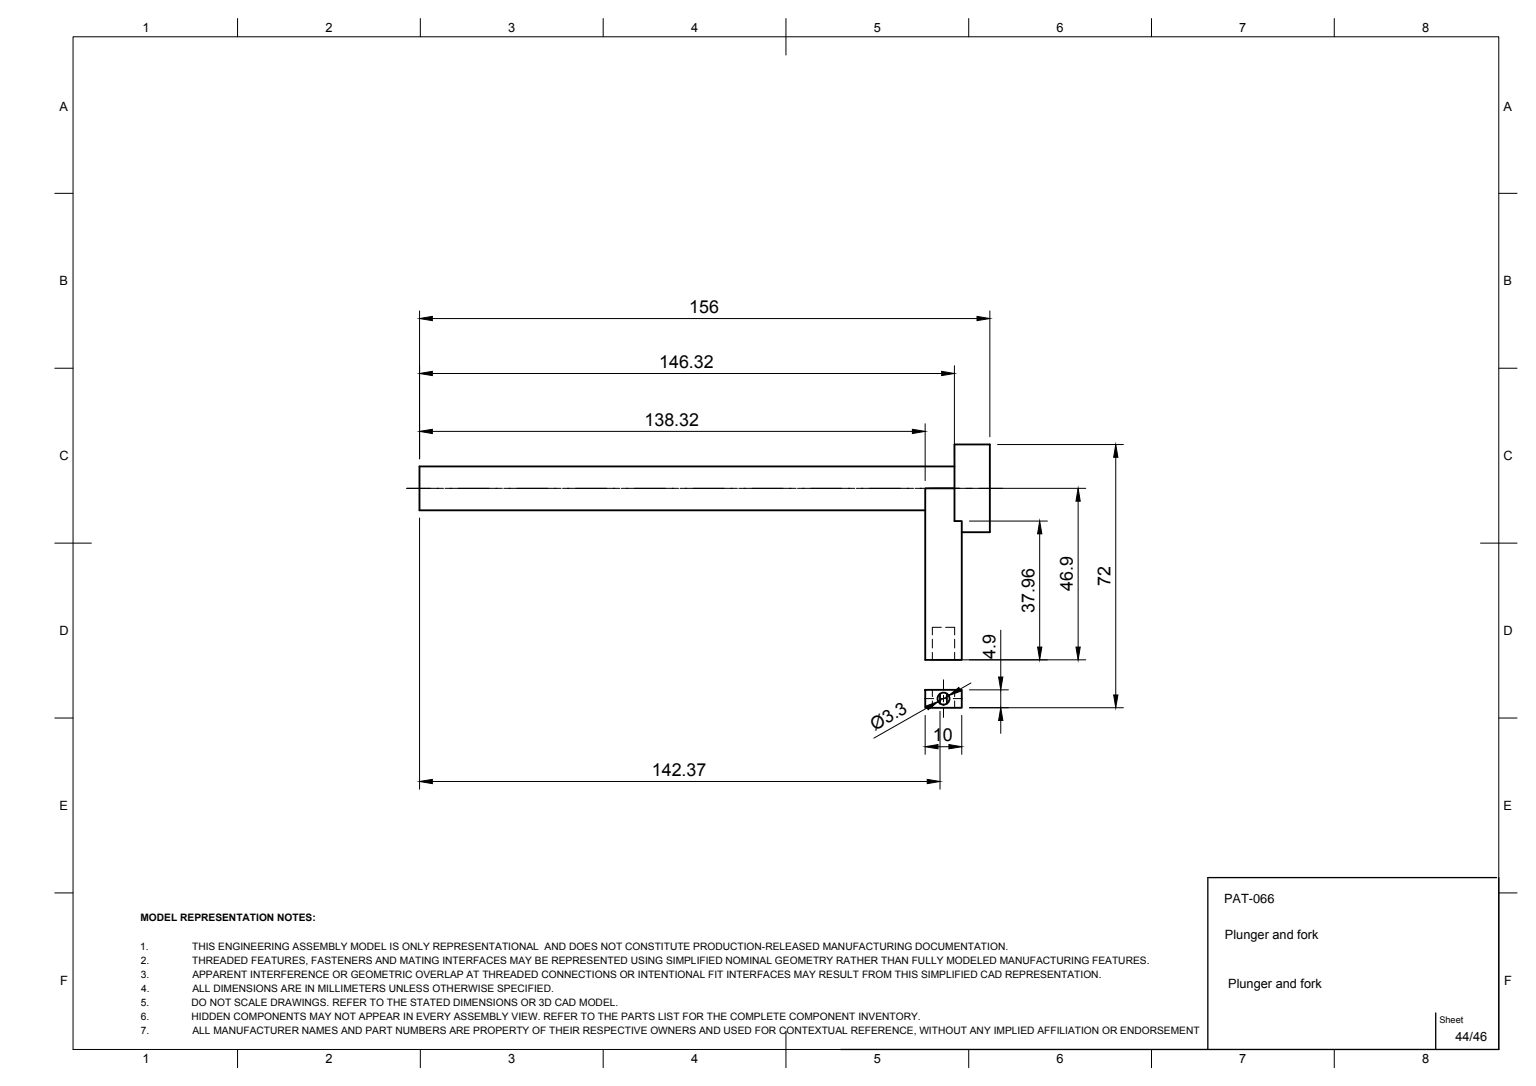
ISO-10303-21;
HEADER;
/* Generated by software containing ST-Developer
 * from STEP Tools, Inc. (www.steptools.com) 
 */

FILE_DESCRIPTION(
/* description */ ('Lever-operated bar clamp (toggle)'),
/* implementation_level */ '2;1');

FILE_NAME(
/* name */ 'Plunger and fork.step',
/* time_stamp */ '2026-10-28T03:25:02-07:00',
/* author */ (''),
/* organization */ (''),
/* preprocessor_version */ 'ST-DEVELOPER v20.2',
/* originating_system */ 'Autodesk Translation Framework v15.17.0.0',
/* authorisation */ '');

FILE_SCHEMA (('AUTOMOTIVE_DESIGN { 1 0 10303 214 3 1 1 }'));
ENDSEC;

DATA;
#10=MECHANICAL_DESIGN_GEOMETRIC_PRESENTATION_REPRESENTATION('',(#452,#453),#12413);
#285=B_SPLINE_CURVE_WITH_KNOTS('',3,(#12174,#12175,#12176,#12177,#12178,
#12179,#12180,#12181,#12182,#12183),.UNSPECIFIED.,.F.,.F.,(4,2,2,2,4),(0.66642709076087,
0.700624974512804,0.764181514210609,0.827738053908413,0.861935937660348),
 .UNSPECIFIED.);
#286=B_SPLINE_CURVE_WITH_KNOTS('',3,(#12191,#12192,#12193,#12194,#12195,
#12196,#12197,#12198,#12199,#12200),.UNSPECIFIED.,.F.,.F.,(4,2,2,2,4),(0.156972747953797,
0.191170631705732,0.254727171403536,0.318283711101341,0.352481594853276),
 .UNSPECIFIED.);
#368=SHAPE_REPRESENTATION_RELATIONSHIP('SRR','None',#12612,#406);
#406=ADVANCED_BREP_SHAPE_REPRESENTATION('',(#495,#496),#12409);
#452=STYLED_ITEM('',(#12883),#495);
#453=STYLED_ITEM('',(#12883),#496);
#495=MANIFOLD_SOLID_BREP('Body1',#6615);
#496=MANIFOLD_SOLID_BREP('Body2',#6616);
#644=FACE_BOUND('',#1803,.T.);
#645=FACE_BOUND('',#1819,.T.);
#646=FACE_BOUND('',#1821,.T.);
#647=FACE_BOUND('',#1826,.T.);
#648=FACE_BOUND('',#1828,.T.);
#855=PLANE('',#7817);
#856=PLANE('',#7818);
#857=PLANE('',#7819);
#858=PLANE('',#7820);
#859=PLANE('',#7822);
#860=PLANE('',#7823);
#861=PLANE('',#7824);
#862=PLANE('',#7825);
#863=PLANE('',#7830);
#864=PLANE('',#7835);
#865=PLANE('',#7836);
#866=PLANE('',#7837);
#867=PLANE('',#7843);
#868=PLANE('',#7847);
#869=PLANE('',#7848);
#870=PLANE('',#7849);
#871=PLANE('',#7850);
#872=PLANE('',#7851);
#873=PLANE('',#7852);
#1250=FACE_OUTER_BOUND('',#1800,.T.);
#1251=FACE_OUTER_BOUND('',#1801,.T.);
#1252=FACE_OUTER_BOUND('',#1802,.T.);
#1253=FACE_OUTER_BOUND('',#1804,.T.);
#1254=FACE_OUTER_BOUND('',#1805,.T.);
#1255=FACE_OUTER_BOUND('',#1806,.T.);
#1256=FACE_OUTER_BOUND('',#1807,.T.);
#1257=FACE_OUTER_BOUND('',#1808,.T.);
#1258=FACE_OUTER_BOUND('',#1809,.T.);
#1259=FACE_OUTER_BOUND('',#1810,.T.);
#1260=FACE_OUTER_BOUND('',#1811,.T.);
#1261=FACE_OUTER_BOUND('',#1812,.T.);
#1262=FACE_OUTER_BOUND('',#1813,.T.);
#1263=FACE_OUTER_BOUND('',#1814,.T.);
#1264=FACE_OUTER_BOUND('',#1815,.T.);
#1265=FACE_OUTER_BOUND('',#1816,.T.);
#1266=FACE_OUTER_BOUND('',#1817,.T.);
#1267=FACE_OUTER_BOUND('',#1818,.T.);
#1268=FACE_OUTER_BOUND('',#1820,.T.);
#1269=FACE_OUTER_BOUND('',#1822,.T.);
#1270=FACE_OUTER_BOUND('',#1823,.T.);
#1271=FACE_OUTER_BOUND('',#1824,.T.);
#1272=FACE_OUTER_BOUND('',#1825,.T.);
#1273=FACE_OUTER_BOUND('',#1827,.T.);
#1800=EDGE_LOOP('',(#5853,#5854,#5855,#5856));
#1801=EDGE_LOOP('',(#5857));
#1802=EDGE_LOOP('',(#5858,#5859,#5860,#5861));
#1803=EDGE_LOOP('',(#5862));
#1804=EDGE_LOOP('',(#5863,#5864,#5865,#5866,#5867,#5868));
#1805=EDGE_LOOP('',(#5869,#5870,#5871,#5872));
#1806=EDGE_LOOP('',(#5873,#5874,#5875,#5876,#5877,#5878));
#1807=EDGE_LOOP('',(#5879,#5880,#5881,#5882));
#1808=EDGE_LOOP('',(#5883,#5884,#5885,#5886));
#1809=EDGE_LOOP('',(#5887,#5888,#5889,#5890,#5891,#5892));
#1810=EDGE_LOOP('',(#5893,#5894,#5895,#5896,#5897,#5898,#5899));
#1811=EDGE_LOOP('',(#5900,#5901,#5902,#5903,#5904,#5905,#5906));
#1812=EDGE_LOOP('',(#5907,#5908,#5909,#5910,#5911,#5912,#5913,#5914));
#1813=EDGE_LOOP('',(#5915));
#1814=EDGE_LOOP('',(#5916));
#1815=EDGE_LOOP('',(#5917,#5918));
#1816=EDGE_LOOP('',(#5919,#5920,#5921,#5922,#5923,#5924,#5925,#5926));
#1817=EDGE_LOOP('',(#5927,#5928,#5929));
#1818=EDGE_LOOP('',(#5930,#5931,#5932,#5933));
#1819=EDGE_LOOP('',(#5934,#5935,#5936,#5937));
#1820=EDGE_LOOP('',(#5938,#5939,#5940,#5941));
#1821=EDGE_LOOP('',(#5942));
#1822=EDGE_LOOP('',(#5943,#5944,#5945,#5946));
#1823=EDGE_LOOP('',(#5947,#5948,#5949,#5950));
#1824=EDGE_LOOP('',(#5951,#5952,#5953,#5954));
#1825=EDGE_LOOP('',(#5955,#5956,#5957,#5958));
#1826=EDGE_LOOP('',(#5959));
#1827=EDGE_LOOP('',(#5960,#5961,#5962,#5963));
#1828=EDGE_LOOP('',(#5964));
#2229=LINE('',#12104,#2670);
#2230=LINE('',#12110,#2671);
#2231=LINE('',#12112,#2672);
#2232=LINE('',#12114,#2673);
#2233=LINE('',#12115,#2674);
#2234=LINE('',#12118,#2675);
#2235=LINE('',#12120,#2676);
#2236=LINE('',#12122,#2677);
#2237=LINE('',#12124,#2678);
#2238=LINE('',#12125,#2679);
#2239=LINE('',#12128,#2680);
#2240=LINE('',#12132,#2681);
#2241=LINE('',#12134,#2682);
#2242=LINE('',#12136,#2683);
#2243=LINE('',#12137,#2684);
#2244=LINE('',#12141,#2685);
#2245=LINE('',#12142,#2686);
#2246=LINE('',#12143,#2687);
#2247=LINE('',#12146,#2688);
#2248=LINE('',#12148,#2689);
#2249=LINE('',#12149,#2690);
#2250=LINE('',#12155,#2691);
#2251=LINE('',#12163,#2692);
#2252=LINE('',#12170,#2693);
#2253=LINE('',#12187,#2694);
#2254=LINE('',#12202,#2695);
#2255=LINE('',#12207,#2696);
#2256=LINE('',#12212,#2697);
#2257=LINE('',#12214,#2698);
#2258=LINE('',#12216,#2699);
#2259=LINE('',#12217,#2700);
#2260=LINE('',#12221,#2701);
#2261=LINE('',#12222,#2702);
#2262=LINE('',#12223,#2703);
#2263=LINE('',#12226,#2704);
#2264=LINE('',#12227,#2705);
#2265=LINE('',#12230,#2706);
#2266=LINE('',#12231,#2707);
#2267=LINE('',#12233,#2708);
#2670=VECTOR('',#9826,0.305);
#2671=VECTOR('',#9833,1.);
#2672=VECTOR('',#9834,1.);
#2673=VECTOR('',#9835,1.);
#2674=VECTOR('',#9836,1.);
#2675=VECTOR('',#9839,1.);
#2676=VECTOR('',#9840,1.);
#2677=VECTOR('',#9841,1.);
#2678=VECTOR('',#9842,1.);
#2679=VECTOR('',#9843,1.);
#2680=VECTOR('',#9846,1.);
#2681=VECTOR('',#9851,1.);
#2682=VECTOR('',#9852,1.);
#2683=VECTOR('',#9853,1.);
#2684=VECTOR('',#9854,1.);
#2685=VECTOR('',#9857,1.);
#2686=VECTOR('',#9858,1.);
#2687=VECTOR('',#9859,1.);
#2688=VECTOR('',#9862,1.);
#2689=VECTOR('',#9863,1.);
#2690=VECTOR('',#9864,1.);
#2691=VECTOR('',#9873,0.6);
#2692=VECTOR('',#9884,1.2);
#2693=VECTOR('',#9893,1.);
#2694=VECTOR('',#9900,0.165);
#2695=VECTOR('',#9907,1.);
#2696=VECTOR('',#9912,0.305);
#2697=VECTOR('',#9917,1.);
#2698=VECTOR('',#9918,1.);
#2699=VECTOR('',#9919,1.);
#2700=VECTOR('',#9920,1.);
#2701=VECTOR('',#9923,1.);
#2702=VECTOR('',#9924,1.);
#2703=VECTOR('',#9925,1.);
#2704=VECTOR('',#9928,1.);
#2705=VECTOR('',#9929,1.);
#2706=VECTOR('',#9932,1.);
#2707=VECTOR('',#9933,1.);
#2708=VECTOR('',#9936,1.);
#3049=CIRCLE('',#7815,0.305);
#3050=CIRCLE('',#7816,0.305);
#3051=CIRCLE('',#7821,1.2);
#3052=CIRCLE('',#7826,0.6);
#3053=CIRCLE('',#7828,0.6);
#3054=CIRCLE('',#7829,0.6);
#3055=CIRCLE('',#7831,1.2);
#3056=CIRCLE('',#7832,1.2);
#3057=CIRCLE('',#7834,1.2);
#3058=CIRCLE('',#7838,0.165);
#3059=CIRCLE('',#7840,0.165);
#3060=CIRCLE('',#7841,0.165);
#3061=CIRCLE('',#7842,0.165);
#3062=CIRCLE('',#7845,0.305);
#3063=CIRCLE('',#7846,0.305);
#3556=VERTEX_POINT('',#12101);
#3557=VERTEX_POINT('',#12103);
#3558=VERTEX_POINT('',#12108);
#3559=VERTEX_POINT('',#12109);
#3560=VERTEX_POINT('',#12111);
#3561=VERTEX_POINT('',#12113);
#3562=VERTEX_POINT('',#12117);
#3563=VERTEX_POINT('',#12119);
#3564=VERTEX_POINT('',#12121);
#3565=VERTEX_POINT('',#12123);
#3566=VERTEX_POINT('',#12127);
#3567=VERTEX_POINT('',#12131);
#3568=VERTEX_POINT('',#12133);
#3569=VERTEX_POINT('',#12135);
#3570=VERTEX_POINT('',#12139);
#3571=VERTEX_POINT('',#12140);
#3572=VERTEX_POINT('',#12145);
#3573=VERTEX_POINT('',#12147);
#3574=VERTEX_POINT('',#12153);
#3575=VERTEX_POINT('',#12158);
#3576=VERTEX_POINT('',#12162);
#3577=VERTEX_POINT('',#12168);
#3578=VERTEX_POINT('',#12169);
#3579=VERTEX_POINT('',#12173);
#3580=VERTEX_POINT('',#12184);
#3581=VERTEX_POINT('',#12186);
#3582=VERTEX_POINT('',#12189);
#3583=VERTEX_POINT('',#12204);
#3584=VERTEX_POINT('',#12206);
#3585=VERTEX_POINT('',#12210);
#3586=VERTEX_POINT('',#12211);
#3587=VERTEX_POINT('',#12213);
#3588=VERTEX_POINT('',#12215);
#3589=VERTEX_POINT('',#12219);
#3590=VERTEX_POINT('',#12220);
#3591=VERTEX_POINT('',#12225);
#3592=VERTEX_POINT('',#12229);
#4331=EDGE_CURVE('',#3556,#3556,#3049,.T.);
#4332=EDGE_CURVE('',#3556,#3557,#2229,.T.);
#4333=EDGE_CURVE('',#3557,#3557,#3050,.T.);
#4334=EDGE_CURVE('',#3558,#3559,#2230,.T.);
#4335=EDGE_CURVE('',#3560,#3558,#2231,.T.);
#4336=EDGE_CURVE('',#3561,#3560,#2232,.T.);
#4337=EDGE_CURVE('',#3559,#3561,#2233,.T.);
#4338=EDGE_CURVE('',#3560,#3562,#2234,.T.);
#4339=EDGE_CURVE('',#3563,#3562,#2235,.T.);
#4340=EDGE_CURVE('',#3564,#3563,#2236,.T.);
#4341=EDGE_CURVE('',#3564,#3565,#2237,.T.);
#4342=EDGE_CURVE('',#3561,#3565,#2238,.T.);
#4343=EDGE_CURVE('',#3566,#3558,#2239,.T.);
#4344=EDGE_CURVE('',#3562,#3566,#3051,.T.);
#4345=EDGE_CURVE('',#3567,#3559,#2240,.T.);
#4346=EDGE_CURVE('',#3568,#3567,#2241,.T.);
#4347=EDGE_CURVE('',#3569,#3568,#2242,.T.);
#4348=EDGE_CURVE('',#3566,#3569,#2243,.T.);
#4349=EDGE_CURVE('',#3570,#3571,#2244,.T.);
#4350=EDGE_CURVE('',#3565,#3570,#2245,.T.);
#4351=EDGE_CURVE('',#3571,#3564,#2246,.T.);
#4352=EDGE_CURVE('',#3568,#3572,#2247,.T.);
#4353=EDGE_CURVE('',#3573,#3567,#2248,.T.);
#4354=EDGE_CURVE('',#3572,#3573,#2249,.T.);
#4355=EDGE_CURVE('',#3573,#3570,#3052,.T.);
#4356=EDGE_CURVE('',#3574,#3574,#3053,.T.);
#4357=EDGE_CURVE('',#3574,#3573,#2250,.T.);
#4358=EDGE_CURVE('',#3571,#3572,#3054,.T.);
#4359=EDGE_CURVE('',#3563,#3575,#3055,.T.);
#4360=EDGE_CURVE('',#3575,#3569,#3056,.T.);
#4361=EDGE_CURVE('',#3575,#3576,#2251,.T.);
#4362=EDGE_CURVE('',#3576,#3576,#3057,.T.);
#4363=EDGE_CURVE('',#3577,#3578,#2252,.T.);
#4364=EDGE_CURVE('',#3577,#3578,#3058,.T.);
#4365=EDGE_CURVE('',#3579,#3577,#285,.T.);
#4366=EDGE_CURVE('',#3580,#3579,#3059,.T.);
#4367=EDGE_CURVE('',#3580,#3581,#2253,.T.);
#4368=EDGE_CURVE('',#3581,#3581,#3060,.T.);
#4369=EDGE_CURVE('',#3582,#3580,#3061,.T.);
#4370=EDGE_CURVE('',#3578,#3582,#286,.T.);
#4371=EDGE_CURVE('',#3582,#3579,#2254,.T.);
#4372=EDGE_CURVE('',#3583,#3583,#3062,.T.);
#4373=EDGE_CURVE('',#3583,#3584,#2255,.T.);
#4374=EDGE_CURVE('',#3584,#3584,#3063,.T.);
#4375=EDGE_CURVE('',#3585,#3586,#2256,.T.);
#4376=EDGE_CURVE('',#3586,#3587,#2257,.T.);
#4377=EDGE_CURVE('',#3588,#3587,#2258,.T.);
#4378=EDGE_CURVE('',#3585,#3588,#2259,.T.);
#4379=EDGE_CURVE('',#3589,#3590,#2260,.T.);
#4380=EDGE_CURVE('',#3590,#3585,#2261,.T.);
#4381=EDGE_CURVE('',#3589,#3588,#2262,.T.);
#4382=EDGE_CURVE('',#3591,#3589,#2263,.T.);
#4383=EDGE_CURVE('',#3587,#3591,#2264,.T.);
#4384=EDGE_CURVE('',#3590,#3592,#2265,.T.);
#4385=EDGE_CURVE('',#3586,#3592,#2266,.T.);
#4386=EDGE_CURVE('',#3592,#3591,#2267,.T.);
#5853=ORIENTED_EDGE('',*,*,#4331,.F.);
#5854=ORIENTED_EDGE('',*,*,#4332,.T.);
#5855=ORIENTED_EDGE('',*,*,#4333,.T.);
#5856=ORIENTED_EDGE('',*,*,#4332,.F.);
#5857=ORIENTED_EDGE('',*,*,#4333,.F.);
#5858=ORIENTED_EDGE('',*,*,#4334,.F.);
#5859=ORIENTED_EDGE('',*,*,#4335,.F.);
#5860=ORIENTED_EDGE('',*,*,#4336,.F.);
#5861=ORIENTED_EDGE('',*,*,#4337,.F.);
#5862=ORIENTED_EDGE('',*,*,#4331,.T.);
#5863=ORIENTED_EDGE('',*,*,#4336,.T.);
#5864=ORIENTED_EDGE('',*,*,#4338,.T.);
#5865=ORIENTED_EDGE('',*,*,#4339,.F.);
#5866=ORIENTED_EDGE('',*,*,#4340,.F.);
#5867=ORIENTED_EDGE('',*,*,#4341,.T.);
#5868=ORIENTED_EDGE('',*,*,#4342,.F.);
#5869=ORIENTED_EDGE('',*,*,#4335,.T.);
#5870=ORIENTED_EDGE('',*,*,#4343,.F.);
#5871=ORIENTED_EDGE('',*,*,#4344,.F.);
#5872=ORIENTED_EDGE('',*,*,#4338,.F.);
#5873=ORIENTED_EDGE('',*,*,#4334,.T.);
#5874=ORIENTED_EDGE('',*,*,#4345,.F.);
#5875=ORIENTED_EDGE('',*,*,#4346,.F.);
#5876=ORIENTED_EDGE('',*,*,#4347,.F.);
#5877=ORIENTED_EDGE('',*,*,#4348,.F.);
#5878=ORIENTED_EDGE('',*,*,#4343,.T.);
#5879=ORIENTED_EDGE('',*,*,#4349,.F.);
#5880=ORIENTED_EDGE('',*,*,#4350,.F.);
#5881=ORIENTED_EDGE('',*,*,#4341,.F.);
#5882=ORIENTED_EDGE('',*,*,#4351,.F.);
#5883=ORIENTED_EDGE('',*,*,#4352,.F.);
#5884=ORIENTED_EDGE('',*,*,#4346,.T.);
#5885=ORIENTED_EDGE('',*,*,#4353,.F.);
#5886=ORIENTED_EDGE('',*,*,#4354,.F.);
#5887=ORIENTED_EDGE('',*,*,#4337,.T.);
#5888=ORIENTED_EDGE('',*,*,#4342,.T.);
#5889=ORIENTED_EDGE('',*,*,#4350,.T.);
#5890=ORIENTED_EDGE('',*,*,#4355,.F.);
#5891=ORIENTED_EDGE('',*,*,#4353,.T.);
#5892=ORIENTED_EDGE('',*,*,#4345,.T.);
#5893=ORIENTED_EDGE('',*,*,#4356,.F.);
#5894=ORIENTED_EDGE('',*,*,#4357,.T.);
#5895=ORIENTED_EDGE('',*,*,#4355,.T.);
#5896=ORIENTED_EDGE('',*,*,#4349,.T.);
#5897=ORIENTED_EDGE('',*,*,#4358,.T.);
#5898=ORIENTED_EDGE('',*,*,#4354,.T.);
#5899=ORIENTED_EDGE('',*,*,#4357,.F.);
#5900=ORIENTED_EDGE('',*,*,#4347,.T.);
#5901=ORIENTED_EDGE('',*,*,#4352,.T.);
#5902=ORIENTED_EDGE('',*,*,#4358,.F.);
#5903=ORIENTED_EDGE('',*,*,#4351,.T.);
#5904=ORIENTED_EDGE('',*,*,#4340,.T.);
#5905=ORIENTED_EDGE('',*,*,#4359,.T.);
#5906=ORIENTED_EDGE('',*,*,#4360,.T.);
#5907=ORIENTED_EDGE('',*,*,#4348,.T.);
#5908=ORIENTED_EDGE('',*,*,#4360,.F.);
#5909=ORIENTED_EDGE('',*,*,#4361,.T.);
#5910=ORIENTED_EDGE('',*,*,#4362,.T.);
#5911=ORIENTED_EDGE('',*,*,#4361,.F.);
#5912=ORIENTED_EDGE('',*,*,#4359,.F.);
#5913=ORIENTED_EDGE('',*,*,#4339,.T.);
#5914=ORIENTED_EDGE('',*,*,#4344,.T.);
#5915=ORIENTED_EDGE('',*,*,#4362,.F.);
#5916=ORIENTED_EDGE('',*,*,#4356,.T.);
#5917=ORIENTED_EDGE('',*,*,#4363,.F.);
#5918=ORIENTED_EDGE('',*,*,#4364,.T.);
#5919=ORIENTED_EDGE('',*,*,#4365,.F.);
#5920=ORIENTED_EDGE('',*,*,#4366,.F.);
#5921=ORIENTED_EDGE('',*,*,#4367,.T.);
#5922=ORIENTED_EDGE('',*,*,#4368,.F.);
#5923=ORIENTED_EDGE('',*,*,#4367,.F.);
#5924=ORIENTED_EDGE('',*,*,#4369,.F.);
#5925=ORIENTED_EDGE('',*,*,#4370,.F.);
#5926=ORIENTED_EDGE('',*,*,#4364,.F.);
#5927=ORIENTED_EDGE('',*,*,#4371,.F.);
#5928=ORIENTED_EDGE('',*,*,#4369,.T.);
#5929=ORIENTED_EDGE('',*,*,#4366,.T.);
#5930=ORIENTED_EDGE('',*,*,#4372,.F.);
#5931=ORIENTED_EDGE('',*,*,#4373,.T.);
#5932=ORIENTED_EDGE('',*,*,#4374,.F.);
#5933=ORIENTED_EDGE('',*,*,#4373,.F.);
#5934=ORIENTED_EDGE('',*,*,#4370,.T.);
#5935=ORIENTED_EDGE('',*,*,#4371,.T.);
#5936=ORIENTED_EDGE('',*,*,#4365,.T.);
#5937=ORIENTED_EDGE('',*,*,#4363,.T.);
#5938=ORIENTED_EDGE('',*,*,#4375,.T.);
#5939=ORIENTED_EDGE('',*,*,#4376,.T.);
#5940=ORIENTED_EDGE('',*,*,#4377,.F.);
#5941=ORIENTED_EDGE('',*,*,#4378,.F.);
#5942=ORIENTED_EDGE('',*,*,#4372,.T.);
#5943=ORIENTED_EDGE('',*,*,#4379,.T.);
#5944=ORIENTED_EDGE('',*,*,#4380,.T.);
#5945=ORIENTED_EDGE('',*,*,#4378,.T.);
#5946=ORIENTED_EDGE('',*,*,#4381,.F.);
#5947=ORIENTED_EDGE('',*,*,#4382,.T.);
#5948=ORIENTED_EDGE('',*,*,#4381,.T.);
#5949=ORIENTED_EDGE('',*,*,#4377,.T.);
#5950=ORIENTED_EDGE('',*,*,#4383,.T.);
#5951=ORIENTED_EDGE('',*,*,#4384,.T.);
#5952=ORIENTED_EDGE('',*,*,#4385,.F.);
#5953=ORIENTED_EDGE('',*,*,#4375,.F.);
#5954=ORIENTED_EDGE('',*,*,#4380,.F.);
#5955=ORIENTED_EDGE('',*,*,#4386,.T.);
#5956=ORIENTED_EDGE('',*,*,#4383,.F.);
#5957=ORIENTED_EDGE('',*,*,#4376,.F.);
#5958=ORIENTED_EDGE('',*,*,#4385,.T.);
#5959=ORIENTED_EDGE('',*,*,#4368,.T.);
#5960=ORIENTED_EDGE('',*,*,#4379,.F.);
#5961=ORIENTED_EDGE('',*,*,#4382,.F.);
#5962=ORIENTED_EDGE('',*,*,#4386,.F.);
#5963=ORIENTED_EDGE('',*,*,#4384,.F.);
#5964=ORIENTED_EDGE('',*,*,#4374,.T.);
#6154=CYLINDRICAL_SURFACE('',#7814,0.305);
#6155=CYLINDRICAL_SURFACE('',#7827,0.6);
#6156=CYLINDRICAL_SURFACE('',#7833,1.2);
#6157=CYLINDRICAL_SURFACE('',#7839,0.165);
#6158=CYLINDRICAL_SURFACE('',#7844,0.305);
#6525=ADVANCED_FACE('',(#1250),#6154,.F.);
#6526=ADVANCED_FACE('',(#1251),#855,.F.);
#6527=ADVANCED_FACE('',(#1252,#644),#856,.F.);
#6528=ADVANCED_FACE('',(#1253),#857,.T.);
#6529=ADVANCED_FACE('',(#1254),#858,.F.);
#6530=ADVANCED_FACE('',(#1255),#859,.T.);
#6531=ADVANCED_FACE('',(#1256),#860,.T.);
#6532=ADVANCED_FACE('',(#1257),#861,.T.);
#6533=ADVANCED_FACE('',(#1258),#862,.T.);
#6534=ADVANCED_FACE('',(#1259),#6155,.T.);
#6535=ADVANCED_FACE('',(#1260),#863,.T.);
#6536=ADVANCED_FACE('',(#1261),#6156,.T.);
#6537=ADVANCED_FACE('',(#1262),#864,.F.);
#6538=ADVANCED_FACE('',(#1263),#865,.T.);
#6539=ADVANCED_FACE('',(#1264),#866,.T.);
#6540=ADVANCED_FACE('',(#1265),#6157,.F.);
#6541=ADVANCED_FACE('',(#1266),#867,.T.);
#6542=ADVANCED_FACE('',(#1267,#645),#6158,.F.);
#6543=ADVANCED_FACE('',(#1268,#646),#868,.T.);
#6544=ADVANCED_FACE('',(#1269),#869,.T.);
#6545=ADVANCED_FACE('',(#1270),#870,.T.);
#6546=ADVANCED_FACE('',(#1271),#871,.F.);
#6547=ADVANCED_FACE('',(#1272,#647),#872,.T.);
#6548=ADVANCED_FACE('',(#1273,#648),#873,.T.);
#6615=CLOSED_SHELL('',(#6525,#6526,#6527,#6528,#6529,#6530,#6531,#6532,
#6533,#6534,#6535,#6536,#6537,#6538));
#6616=CLOSED_SHELL('',(#6539,#6540,#6541,#6542,#6543,#6544,#6545,#6546,
#6547,#6548));
#7813=AXIS2_PLACEMENT_3D('',#12099,#9820,#9821);
#7814=AXIS2_PLACEMENT_3D('',#12100,#9822,#9823);
#7815=AXIS2_PLACEMENT_3D('',#12102,#9824,#9825);
#7816=AXIS2_PLACEMENT_3D('',#12105,#9827,#9828);
#7817=AXIS2_PLACEMENT_3D('',#12106,#9829,#9830);
#7818=AXIS2_PLACEMENT_3D('',#12107,#9831,#9832);
#7819=AXIS2_PLACEMENT_3D('',#12116,#9837,#9838);
#7820=AXIS2_PLACEMENT_3D('',#12126,#9844,#9845);
#7821=AXIS2_PLACEMENT_3D('',#12129,#9847,#9848);
#7822=AXIS2_PLACEMENT_3D('',#12130,#9849,#9850);
#7823=AXIS2_PLACEMENT_3D('',#12138,#9855,#9856);
#7824=AXIS2_PLACEMENT_3D('',#12144,#9860,#9861);
#7825=AXIS2_PLACEMENT_3D('',#12150,#9865,#9866);
#7826=AXIS2_PLACEMENT_3D('',#12151,#9867,#9868);
#7827=AXIS2_PLACEMENT_3D('',#12152,#9869,#9870);
#7828=AXIS2_PLACEMENT_3D('',#12154,#9871,#9872);
#7829=AXIS2_PLACEMENT_3D('',#12156,#9874,#9875);
#7830=AXIS2_PLACEMENT_3D('',#12157,#9876,#9877);
#7831=AXIS2_PLACEMENT_3D('',#12159,#9878,#9879);
#7832=AXIS2_PLACEMENT_3D('',#12160,#9880,#9881);
#7833=AXIS2_PLACEMENT_3D('',#12161,#9882,#9883);
#7834=AXIS2_PLACEMENT_3D('',#12164,#9885,#9886);
#7835=AXIS2_PLACEMENT_3D('',#12165,#9887,#9888);
#7836=AXIS2_PLACEMENT_3D('',#12166,#9889,#9890);
#7837=AXIS2_PLACEMENT_3D('',#12167,#9891,#9892);
#7838=AXIS2_PLACEMENT_3D('',#12171,#9894,#9895);
#7839=AXIS2_PLACEMENT_3D('',#12172,#9896,#9897);
#7840=AXIS2_PLACEMENT_3D('',#12185,#9898,#9899);
#7841=AXIS2_PLACEMENT_3D('',#12188,#9901,#9902);
#7842=AXIS2_PLACEMENT_3D('',#12190,#9903,#9904);
#7843=AXIS2_PLACEMENT_3D('',#12201,#9905,#9906);
#7844=AXIS2_PLACEMENT_3D('',#12203,#9908,#9909);
#7845=AXIS2_PLACEMENT_3D('',#12205,#9910,#9911);
#7846=AXIS2_PLACEMENT_3D('',#12208,#9913,#9914);
#7847=AXIS2_PLACEMENT_3D('',#12209,#9915,#9916);
#7848=AXIS2_PLACEMENT_3D('',#12218,#9921,#9922);
#7849=AXIS2_PLACEMENT_3D('',#12224,#9926,#9927);
#7850=AXIS2_PLACEMENT_3D('',#12228,#9930,#9931);
#7851=AXIS2_PLACEMENT_3D('',#12232,#9934,#9935);
#7852=AXIS2_PLACEMENT_3D('',#12234,#9937,#9938);
#9820=DIRECTION('axis',(0.,0.,1.));
#9821=DIRECTION('refdir',(1.,0.,0.));
#9822=DIRECTION('center_axis',(0.,1.,0.));
#9823=DIRECTION('ref_axis',(1.,0.,0.));
#9824=DIRECTION('center_axis',(0.,1.,0.));
#9825=DIRECTION('ref_axis',(1.,0.,0.));
#9826=DIRECTION('',(0.,1.,0.));
#9827=DIRECTION('center_axis',(0.,1.,0.));
#9828=DIRECTION('ref_axis',(1.,0.,0.));
#9829=DIRECTION('center_axis',(0.,1.,0.));
#9830=DIRECTION('ref_axis',(1.,0.,0.));
#9831=DIRECTION('center_axis',(0.,1.,0.));
#9832=DIRECTION('ref_axis',(0.,0.,1.));
#9833=DIRECTION('',(0.,0.,1.));
#9834=DIRECTION('',(-1.,0.,0.));
#9835=DIRECTION('',(0.,0.,-1.));
#9836=DIRECTION('',(1.,0.,0.));
#9837=DIRECTION('center_axis',(1.,0.,0.));
#9838=DIRECTION('ref_axis',(0.,1.,0.));
#9839=DIRECTION('',(0.,1.,0.));
#9840=DIRECTION('',(0.,0.,-1.));
#9841=DIRECTION('',(0.,-1.,0.));
#9842=DIRECTION('',(0.,0.,1.));
#9843=DIRECTION('',(0.,1.,0.));
#9844=DIRECTION('center_axis',(0.,0.,1.));
#9845=DIRECTION('ref_axis',(1.,0.,0.));
#9846=DIRECTION('',(0.,-1.,0.));
#9847=DIRECTION('center_axis',(0.,0.,-1.));
#9848=DIRECTION('ref_axis',(1.,0.,0.));
#9849=DIRECTION('center_axis',(-1.,0.,0.));
#9850=DIRECTION('ref_axis',(0.,-1.,0.));
#9851=DIRECTION('',(0.,-1.,0.));
#9852=DIRECTION('',(0.,0.,1.));
#9853=DIRECTION('',(0.,1.,0.));
#9854=DIRECTION('',(0.,0.,1.));
#9855=DIRECTION('center_axis',(0.,1.,0.));
#9856=DIRECTION('ref_axis',(-1.,0.,0.));
#9857=DIRECTION('',(0.,0.,-1.));
#9858=DIRECTION('',(-1.,0.,0.));
#9859=DIRECTION('',(1.,0.,0.));
#9860=DIRECTION('center_axis',(0.,1.,0.));
#9861=DIRECTION('ref_axis',(-1.,0.,0.));
#9862=DIRECTION('',(1.,0.,0.));
#9863=DIRECTION('',(-1.,0.,0.));
#9864=DIRECTION('',(0.,0.,1.));
#9865=DIRECTION('center_axis',(0.,0.,1.));
#9866=DIRECTION('ref_axis',(1.,0.,0.));
#9867=DIRECTION('center_axis',(0.,0.,1.));
#9868=DIRECTION('ref_axis',(1.,0.,0.));
#9869=DIRECTION('center_axis',(0.,0.,1.));
#9870=DIRECTION('ref_axis',(1.,0.,0.));
#9871=DIRECTION('center_axis',(0.,0.,1.));
#9872=DIRECTION('ref_axis',(1.,0.,0.));
#9873=DIRECTION('',(0.,0.,-1.));
#9874=DIRECTION('center_axis',(0.,0.,1.));
#9875=DIRECTION('ref_axis',(1.,0.,0.));
#9876=DIRECTION('center_axis',(0.,0.,1.));
#9877=DIRECTION('ref_axis',(1.,0.,0.));
#9878=DIRECTION('center_axis',(0.,0.,1.));
#9879=DIRECTION('ref_axis',(1.,0.,0.));
#9880=DIRECTION('center_axis',(0.,0.,1.));
#9881=DIRECTION('ref_axis',(1.,0.,0.));
#9882=DIRECTION('center_axis',(0.,0.,1.));
#9883=DIRECTION('ref_axis',(1.,0.,0.));
#9884=DIRECTION('',(0.,0.,-1.));
#9885=DIRECTION('center_axis',(0.,0.,1.));
#9886=DIRECTION('ref_axis',(1.,0.,0.));
#9887=DIRECTION('center_axis',(0.,0.,1.));
#9888=DIRECTION('ref_axis',(1.,0.,0.));
#9889=DIRECTION('center_axis',(0.,0.,1.));
#9890=DIRECTION('ref_axis',(1.,0.,0.));
#9891=DIRECTION('center_axis',(1.,0.,0.));
#9892=DIRECTION('ref_axis',(0.,0.,-1.));
#9893=DIRECTION('',(0.,1.,0.));
#9894=DIRECTION('center_axis',(1.,0.,0.));
#9895=DIRECTION('ref_axis',(0.,0.,-1.));
#9896=DIRECTION('center_axis',(1.,0.,0.));
#9897=DIRECTION('ref_axis',(0.,0.,-1.));
#9898=DIRECTION('center_axis',(1.,0.,0.));
#9899=DIRECTION('ref_axis',(0.,0.,-1.));
#9900=DIRECTION('',(1.,0.,0.));
#9901=DIRECTION('center_axis',(-1.,0.,0.));
#9902=DIRECTION('ref_axis',(0.,0.,-1.));
#9903=DIRECTION('center_axis',(1.,0.,0.));
#9904=DIRECTION('ref_axis',(0.,0.,-1.));
#9905=DIRECTION('center_axis',(1.,0.,0.));
#9906=DIRECTION('ref_axis',(0.,0.,-1.));
#9907=DIRECTION('',(0.,-1.,0.));
#9908=DIRECTION('center_axis',(0.,1.,0.));
#9909=DIRECTION('ref_axis',(1.,0.,0.));
#9910=DIRECTION('center_axis',(0.,1.,0.));
#9911=DIRECTION('ref_axis',(1.,0.,0.));
#9912=DIRECTION('',(0.,1.,0.));
#9913=DIRECTION('center_axis',(0.,-1.,0.));
#9914=DIRECTION('ref_axis',(1.,0.,0.));
#9915=DIRECTION('center_axis',(0.,-1.,0.));
#9916=DIRECTION('ref_axis',(1.,0.,0.));
#9917=DIRECTION('',(1.,0.,0.));
#9918=DIRECTION('',(0.,0.,1.));
#9919=DIRECTION('',(1.,0.,0.));
#9920=DIRECTION('',(0.,0.,1.));
#9921=DIRECTION('center_axis',(-1.,0.,0.));
#9922=DIRECTION('ref_axis',(0.,-1.,0.));
#9923=DIRECTION('',(0.,0.,-1.));
#9924=DIRECTION('',(0.,-1.,0.));
#9925=DIRECTION('',(0.,-1.,0.));
#9926=DIRECTION('center_axis',(0.,0.,1.));
#9927=DIRECTION('ref_axis',(1.,0.,0.));
#9928=DIRECTION('',(-1.,0.,0.));
#9929=DIRECTION('',(0.,1.,0.));
#9930=DIRECTION('center_axis',(0.,0.,1.));
#9931=DIRECTION('ref_axis',(1.,0.,0.));
#9932=DIRECTION('',(1.,0.,0.));
#9933=DIRECTION('',(0.,1.,0.));
#9934=DIRECTION('center_axis',(1.,0.,0.));
#9935=DIRECTION('ref_axis',(0.,1.,0.));
#9936=DIRECTION('',(0.,0.,1.));
#9937=DIRECTION('center_axis',(0.,1.,0.));
#9938=DIRECTION('ref_axis',(1.,0.,0.));
#12099=CARTESIAN_POINT('',(0.,0.,0.));
#12100=CARTESIAN_POINT('Origin',(0.,-6.1,4.668081457105));
#12101=CARTESIAN_POINT('',(-0.305,-4.69,4.668081457105));
#12102=CARTESIAN_POINT('Origin',(0.,-4.69,4.668081457105));
#12103=CARTESIAN_POINT('',(-0.305,-3.8,4.668081457105));
#12104=CARTESIAN_POINT('',(-0.305,-6.1,4.668081457105));
#12105=CARTESIAN_POINT('Origin',(0.,-3.8,4.668081457105));
#12106=CARTESIAN_POINT('Origin',(0.,-3.8,4.668081457105));
#12107=CARTESIAN_POINT('Origin',(0.,-4.69,4.668081457105));
#12108=CARTESIAN_POINT('',(-0.8,-4.69,4.16808146));
#12109=CARTESIAN_POINT('',(-0.8,-4.69,5.16808146));
#12110=CARTESIAN_POINT('',(-0.8,-4.69,4.4180814585525));
#12111=CARTESIAN_POINT('',(0.8,-4.69,4.16808146));
#12112=CARTESIAN_POINT('',(0.,-4.69,4.16808146));
#12113=CARTESIAN_POINT('',(0.8,-4.69,5.16808146));
#12114=CARTESIAN_POINT('',(0.8,-4.69,4.4180814585525));
#12115=CARTESIAN_POINT('',(0.,-4.69,5.16808146));
#12116=CARTESIAN_POINT('Origin',(0.8,-6.,4.16808146));
#12117=CARTESIAN_POINT('',(0.8,-0.894427190999916,4.16808146));
#12118=CARTESIAN_POINT('',(0.8,-6.,4.16808146));
#12119=CARTESIAN_POINT('',(0.8,-0.894427190999916,4.36808146));
#12120=CARTESIAN_POINT('',(0.8,-0.894427190999916,3.4));
#12121=CARTESIAN_POINT('',(0.8,0.,4.36808146));
#12122=CARTESIAN_POINT('',(0.8,-3.,4.36808146));
#12123=CARTESIAN_POINT('',(0.8,0.,5.16808146));
#12124=CARTESIAN_POINT('',(0.8,0.,4.16808146));
#12125=CARTESIAN_POINT('',(0.8,-6.,5.16808146));
#12126=CARTESIAN_POINT('Origin',(0.,-3.,4.16808146));
#12127=CARTESIAN_POINT('',(-0.8,-0.894427190999916,4.16808146));
#12128=CARTESIAN_POINT('',(-0.8,0.,4.16808146));
#12129=CARTESIAN_POINT('Origin',(0.,0.,4.16808146));
#12130=CARTESIAN_POINT('Origin',(-0.8,0.,4.16808146));
#12131=CARTESIAN_POINT('',(-0.8,0.,5.16808146));
#12132=CARTESIAN_POINT('',(-0.8,0.,5.16808146));
#12133=CARTESIAN_POINT('',(-0.8,0.,4.36808146));
#12134=CARTESIAN_POINT('',(-0.8,0.,4.16808146));
#12135=CARTESIAN_POINT('',(-0.8,-0.894427190999916,4.36808146));
#12136=CARTESIAN_POINT('',(-0.8,0.,4.36808146));
#12137=CARTESIAN_POINT('',(-0.8,-0.894427190999916,3.4));
#12138=CARTESIAN_POINT('Origin',(0.8,0.,4.16808146));
#12139=CARTESIAN_POINT('',(0.6,0.,5.16808146));
#12140=CARTESIAN_POINT('',(0.6,0.,4.36808146));
#12141=CARTESIAN_POINT('',(0.6,0.,4.36808146));
#12142=CARTESIAN_POINT('',(0.8,0.,5.16808146));
#12143=CARTESIAN_POINT('',(0.4,0.,4.36808146));
#12144=CARTESIAN_POINT('Origin',(0.8,0.,4.16808146));
#12145=CARTESIAN_POINT('',(-0.6,-7.34788079488412E-17,4.36808146));
#12146=CARTESIAN_POINT('',(0.4,0.,4.36808146));
#12147=CARTESIAN_POINT('',(-0.6,0.,5.16808146));
#12148=CARTESIAN_POINT('',(0.8,0.,5.16808146));
#12149=CARTESIAN_POINT('',(-0.6,0.,4.36808146));
#12150=CARTESIAN_POINT('Origin',(0.,-3.,5.16808146));
#12151=CARTESIAN_POINT('Origin',(0.,0.,5.16808146));
#12152=CARTESIAN_POINT('Origin',(0.,0.,4.36808146));
#12153=CARTESIAN_POINT('',(-0.6,-7.34788079488412E-17,19.));
#12154=CARTESIAN_POINT('Origin',(0.,0.,19.));
#12155=CARTESIAN_POINT('',(-0.6,-7.34788079488412E-17,4.36808146));
#12156=CARTESIAN_POINT('Origin',(0.,0.,4.36808146));
#12157=CARTESIAN_POINT('Origin',(0.,0.,4.36808146));
#12158=CARTESIAN_POINT('',(-1.2,-1.46957615897682E-16,4.36808146));
#12159=CARTESIAN_POINT('Origin',(0.,0.,4.36808146));
#12160=CARTESIAN_POINT('Origin',(0.,0.,4.36808146));
#12161=CARTESIAN_POINT('Origin',(0.,0.,3.4));
#12162=CARTESIAN_POINT('',(-1.2,-1.46957615897682E-16,3.4));
#12163=CARTESIAN_POINT('',(-1.2,-1.46957615897682E-16,3.4));
#12164=CARTESIAN_POINT('Origin',(0.,0.,3.4));
#12165=CARTESIAN_POINT('Origin',(0.,0.,3.4));
#12166=CARTESIAN_POINT('Origin',(0.,0.,19.));
#12167=CARTESIAN_POINT('Origin',(0.29,-5.75,4.668081457105));
#12168=CARTESIAN_POINT('',(0.29,-5.88527749258469,4.57360923896654));
#12169=CARTESIAN_POINT('',(0.29,-5.61472250741531,4.57360923896654));
#12170=CARTESIAN_POINT('',(0.29,-6.1,4.57360923896654));
#12171=CARTESIAN_POINT('Origin',(0.29,-5.75,4.668081457105));
#12172=CARTESIAN_POINT('Origin',(0.29,-5.75,4.668081457105));
#12173=CARTESIAN_POINT('',(0.29,-5.88527749258469,4.76255367524346));
#12174=CARTESIAN_POINT('Ctrl Pts',(0.29,-5.88527749258469,4.76255367524346));
#12175=CARTESIAN_POINT('Ctrl Pts',(0.293078111442152,-5.89187616839667,
4.75310484112255));
#12176=CARTESIAN_POINT('Ctrl Pts',(0.295928845896546,-5.89761208817693,
4.7427508396533));
#12177=CARTESIAN_POINT('Ctrl Pts',(0.302593996394854,-5.91067507972101,
4.71157336496124));
#12178=CARTESIAN_POINT('Ctrl Pts',(0.305,-5.915,4.6892669703376));
#12179=CARTESIAN_POINT('Ctrl Pts',(0.305,-5.915,4.6468959438724));
#12180=CARTESIAN_POINT('Ctrl Pts',(0.302593996394854,-5.91067507972101,
4.62458954924876));
#12181=CARTESIAN_POINT('Ctrl Pts',(0.295928845896546,-5.89761208817693,
4.5934120745567));
#12182=CARTESIAN_POINT('Ctrl Pts',(0.293078111442152,-5.89187616839667,
4.58305807308745));
#12183=CARTESIAN_POINT('Ctrl Pts',(0.29,-5.88527749258469,4.57360923896654));
#12184=CARTESIAN_POINT('',(0.29,-5.75,4.833081457105));
#12185=CARTESIAN_POINT('Origin',(0.29,-5.75,4.668081457105));
#12186=CARTESIAN_POINT('',(0.8,-5.75,4.833081457105));
#12187=CARTESIAN_POINT('',(0.29,-5.75,4.833081457105));
#12188=CARTESIAN_POINT('Origin',(0.8,-5.75,4.668081457105));
#12189=CARTESIAN_POINT('',(0.29,-5.61472250741531,4.76255367524346));
#12190=CARTESIAN_POINT('Origin',(0.29,-5.75,4.668081457105));
#12191=CARTESIAN_POINT('Ctrl Pts',(0.29,-5.61472250741531,4.57360923896654));
#12192=CARTESIAN_POINT('Ctrl Pts',(0.293078111442152,-5.60812383160333,
4.58305807308745));
#12193=CARTESIAN_POINT('Ctrl Pts',(0.295928845896546,-5.60238791182307,
4.5934120745567));
#12194=CARTESIAN_POINT('Ctrl Pts',(0.302593996394854,-5.58932492027899,
4.62458954924876));
#12195=CARTESIAN_POINT('Ctrl Pts',(0.305,-5.585,4.6468959438724));
#12196=CARTESIAN_POINT('Ctrl Pts',(0.305,-5.585,4.6892669703376));
#12197=CARTESIAN_POINT('Ctrl Pts',(0.302593996394854,-5.58932492027899,
4.71157336496124));
#12198=CARTESIAN_POINT('Ctrl Pts',(0.295928845896546,-5.60238791182307,
4.7427508396533));
#12199=CARTESIAN_POINT('Ctrl Pts',(0.293078111442152,-5.60812383160333,
4.75310484112255));
#12200=CARTESIAN_POINT('Ctrl Pts',(0.29,-5.61472250741531,4.76255367524346));
#12201=CARTESIAN_POINT('Origin',(0.29,-5.75,4.668081457105));
#12202=CARTESIAN_POINT('',(0.29,-6.1,4.76255367524346));
#12203=CARTESIAN_POINT('Origin',(0.,-6.1,4.668081457105));
#12204=CARTESIAN_POINT('',(-0.305,-6.,4.668081457105));
#12205=CARTESIAN_POINT('Origin',(0.,-6.,4.668081457105));
#12206=CARTESIAN_POINT('',(-0.305,-5.51,4.668081457105));
#12207=CARTESIAN_POINT('',(-0.305,-6.1,4.668081457105));
#12208=CARTESIAN_POINT('Origin',(0.,-5.51,4.668081457105));
#12209=CARTESIAN_POINT('Origin',(-0.8,-6.,4.16808146));
#12210=CARTESIAN_POINT('',(-0.8,-6.,4.16808146));
#12211=CARTESIAN_POINT('',(0.8,-6.,4.16808146));
#12212=CARTESIAN_POINT('',(-0.8,-6.,4.16808146));
#12213=CARTESIAN_POINT('',(0.8,-6.,5.16808146));
#12214=CARTESIAN_POINT('',(0.8,-6.,4.16808146));
#12215=CARTESIAN_POINT('',(-0.8,-6.,5.16808146));
#12216=CARTESIAN_POINT('',(-0.8,-6.,5.16808146));
#12217=CARTESIAN_POINT('',(-0.8,-6.,4.16808146));
#12218=CARTESIAN_POINT('Origin',(-0.8,0.,4.16808146));
#12219=CARTESIAN_POINT('',(-0.8,-5.51,5.16808146));
#12220=CARTESIAN_POINT('',(-0.8,-5.51,4.16808146));
#12221=CARTESIAN_POINT('',(-0.8,-5.51,4.4180814585525));
#12222=CARTESIAN_POINT('',(-0.8,0.,4.16808146));
#12223=CARTESIAN_POINT('',(-0.8,0.,5.16808146));
#12224=CARTESIAN_POINT('Origin',(0.,-3.,5.16808146));
#12225=CARTESIAN_POINT('',(0.8,-5.51,5.16808146));
#12226=CARTESIAN_POINT('',(0.,-5.51,5.16808146));
#12227=CARTESIAN_POINT('',(0.8,-6.,5.16808146));
#12228=CARTESIAN_POINT('Origin',(0.,-3.,4.16808146));
#12229=CARTESIAN_POINT('',(0.8,-5.51,4.16808146));
#12230=CARTESIAN_POINT('',(0.,-5.51,4.16808146));
#12231=CARTESIAN_POINT('',(0.8,-6.,4.16808146));
#12232=CARTESIAN_POINT('Origin',(0.8,-6.,4.16808146));
#12233=CARTESIAN_POINT('',(0.8,-5.51,4.4180814585525));
#12234=CARTESIAN_POINT('Origin',(0.,-5.51,4.668081457105));
#12363=UNCERTAINTY_MEASURE_WITH_UNIT(LENGTH_MEASURE(0.001),#12414,
'DISTANCE_ACCURACY_VALUE',
'Maximum model space distance between geometric entities at asserted c
onnectivities');
#12367=UNCERTAINTY_MEASURE_WITH_UNIT(LENGTH_MEASURE(0.001),#12414,
'DISTANCE_ACCURACY_VALUE',
'Maximum model space distance between geometric entities at asserted c
onnectivities');
#12409=(
GEOMETRIC_REPRESENTATION_CONTEXT(3)
GLOBAL_UNCERTAINTY_ASSIGNED_CONTEXT((#12363))
GLOBAL_UNIT_ASSIGNED_CONTEXT((#12414,#12416,#12417))
REPRESENTATION_CONTEXT('','3D')
);
#12413=(
GEOMETRIC_REPRESENTATION_CONTEXT(3)
GLOBAL_UNCERTAINTY_ASSIGNED_CONTEXT((#12367))
GLOBAL_UNIT_ASSIGNED_CONTEXT((#12414,#12416,#12417))
REPRESENTATION_CONTEXT('','3D')
);
#12414=(
LENGTH_UNIT()
NAMED_UNIT(*)
SI_UNIT(.CENTI.,.METRE.)
);
#12416=(
NAMED_UNIT(*)
PLANE_ANGLE_UNIT()
SI_UNIT($,.RADIAN.)
);
#12417=(
NAMED_UNIT(*)
SI_UNIT($,.STERADIAN.)
SOLID_ANGLE_UNIT()
);
#12459=SHAPE_DEFINITION_REPRESENTATION(#12559,#12612);
#12559=PRODUCT_DEFINITION_SHAPE('',$,#12658);
#12612=SHAPE_REPRESENTATION('',(#7813),#12409);
#12616=PRODUCT_DEFINITION_CONTEXT('part definition',#12753,'design');
#12658=PRODUCT_DEFINITION('Plunger and fork','Plunger and fork',#12703,
#12616);
#12703=PRODUCT_DEFINITION_FORMATION('',$,#12796);
#12753=APPLICATION_CONTEXT(
'Core Data for Automotive Mechanical Design Process');
#12754=PRODUCT_CONTEXT('part definition',#12753,'mechanical');
#12796=PRODUCT('Plunger and fork','Plunger and fork','Plunger and fork',
(#12754));
#12877=COLOUR_RGB('Off White',0.89,0.88,0.83);
#12878=FILL_AREA_STYLE_COLOUR('',#12877);
#12879=FILL_AREA_STYLE('',(#12878));
#12880=SURFACE_STYLE_FILL_AREA(#12879);
#12881=SURFACE_SIDE_STYLE('',(#12880));
#12882=SURFACE_STYLE_USAGE(.BOTH.,#12881);
#12883=PRESENTATION_STYLE_ASSIGNMENT((#12882));
ENDSEC;
END-ISO-10303-21;
